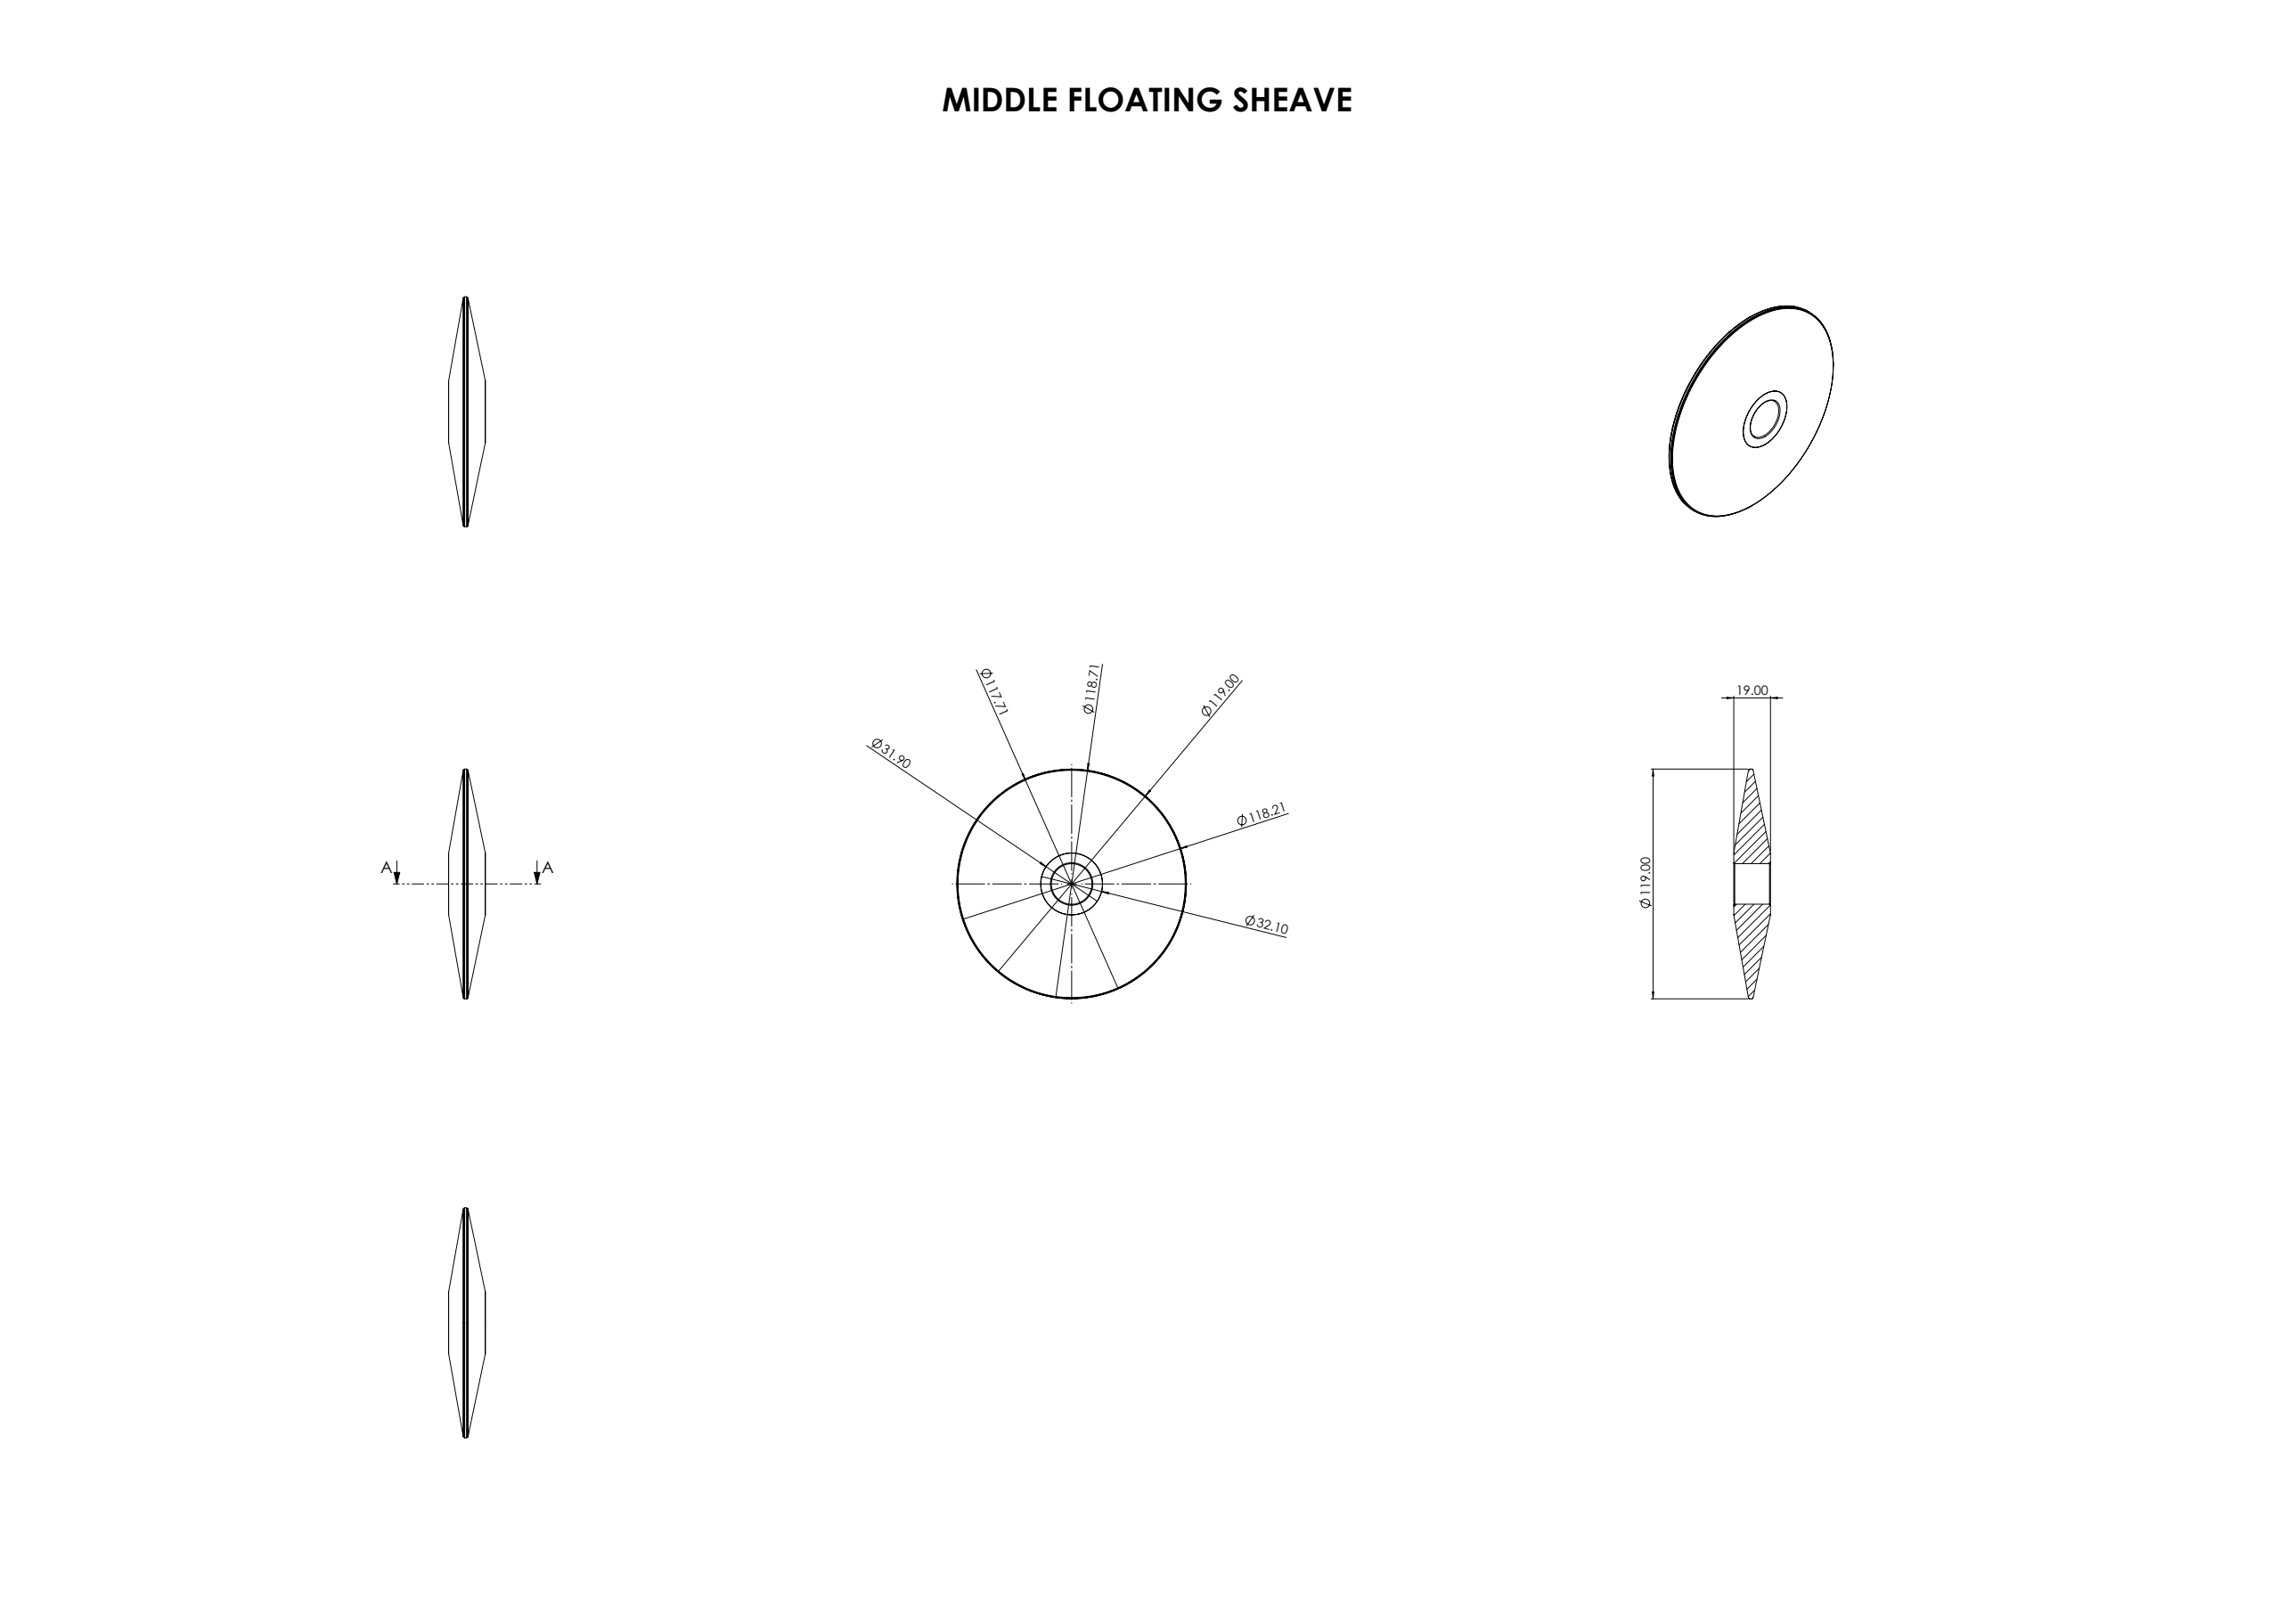
ISO-10303-21;
HEADER;
/* Generated by software containing ST-Developer
 * from STEP Tools, Inc. (www.steptools.com) 
 */

FILE_DESCRIPTION(
/* description */ (''),
/* implementation_level */ '2;1');

FILE_NAME(
/* name */ '02_Middle_Floating_Sheave.step',
/* time_stamp */ '2026-10-24T13:41:11-07:00',
/* author */ (''),
/* organization */ (''),
/* preprocessor_version */ 'ST-DEVELOPER v20.2',
/* originating_system */ 'Autodesk Translation Framework v15.15.0.0',
/* authorisation */ '');

FILE_SCHEMA (('AUTOMOTIVE_DESIGN { 1 0 10303 214 3 1 1 }'));
ENDSEC;

DATA;
#10=MECHANICAL_DESIGN_GEOMETRIC_PRESENTATION_REPRESENTATION('',(#122),#12813);
#81=CONICAL_SURFACE('',#4567,37.5,1.36447243276518);
#82=CONICAL_SURFACE('',#4576,59.25,0.785398163397448);
#83=CONICAL_SURFACE('',#4590,59.25,0.785398163397448);
#84=CONICAL_SURFACE('',#4597,37.5,1.39585880542621);
#102=SHAPE_REPRESENTATION_RELATIONSHIP('SRR','None',#12855,#112);
#112=ADVANCED_BREP_SHAPE_REPRESENTATION('',(#132),#12804);
#122=STYLED_ITEM('',(#12988),#132);
#132=MANIFOLD_SOLID_BREP('Body1',#4385);
#144=FACE_BOUND('',#632,.T.);
#145=FACE_BOUND('',#643,.T.);
#176=PLANE('',#4570);
#177=PLANE('',#4603);
#264=TOROIDAL_SURFACE('',#4562,15.9482352626124,0.5);
#265=TOROIDAL_SURFACE('',#4572,58.7517732660432,0.5);
#266=TOROIDAL_SURFACE('',#4579,59.,0.5);
#267=TOROIDAL_SURFACE('',#4586,59.,0.5);
#268=TOROIDAL_SURFACE('',#4593,58.7578429367487,0.5);
#269=TOROIDAL_SURFACE('',#4600,15.9561537431677,0.5);
#270=TOROIDAL_SURFACE('',#4605,11.,0.5);
#271=TOROIDAL_SURFACE('',#4612,11.,0.5);
#356=FACE_OUTER_BOUND('',#629,.T.);
#357=FACE_OUTER_BOUND('',#630,.T.);
#358=FACE_OUTER_BOUND('',#631,.T.);
#359=FACE_OUTER_BOUND('',#633,.T.);
#360=FACE_OUTER_BOUND('',#634,.T.);
#361=FACE_OUTER_BOUND('',#635,.T.);
#362=FACE_OUTER_BOUND('',#636,.T.);
#363=FACE_OUTER_BOUND('',#637,.T.);
#364=FACE_OUTER_BOUND('',#638,.T.);
#365=FACE_OUTER_BOUND('',#639,.T.);
#366=FACE_OUTER_BOUND('',#640,.T.);
#367=FACE_OUTER_BOUND('',#641,.T.);
#368=FACE_OUTER_BOUND('',#642,.T.);
#369=FACE_OUTER_BOUND('',#644,.T.);
#370=FACE_OUTER_BOUND('',#645,.T.);
#371=FACE_OUTER_BOUND('',#646,.T.);
#629=EDGE_LOOP('',(#2913,#2914,#2915,#2916,#2917));
#630=EDGE_LOOP('',(#2918,#2919,#2920,#2921,#2922,#2923));
#631=EDGE_LOOP('',(#2924));
#632=EDGE_LOOP('',(#2925));
#633=EDGE_LOOP('',(#2926,#2927,#2928,#2929,#2930,#2931));
#634=EDGE_LOOP('',(#2932,#2933,#2934,#2935,#2936,#2937));
#635=EDGE_LOOP('',(#2938,#2939,#2940,#2941,#2942,#2943));
#636=EDGE_LOOP('',(#2944,#2945,#2946,#2947,#2948,#2949));
#637=EDGE_LOOP('',(#2950,#2951,#2952,#2953,#2954,#2955));
#638=EDGE_LOOP('',(#2956,#2957,#2958,#2959,#2960,#2961));
#639=EDGE_LOOP('',(#2962,#2963,#2964,#2965,#2966,#2967));
#640=EDGE_LOOP('',(#2968,#2969,#2970,#2971,#2972,#2973));
#641=EDGE_LOOP('',(#2974,#2975,#2976,#2977,#2978));
#642=EDGE_LOOP('',(#2979));
#643=EDGE_LOOP('',(#2980));
#644=EDGE_LOOP('',(#2981,#2982,#2983,#2984,#2985));
#645=EDGE_LOOP('',(#2986,#2987,#2988,#2989,#2990,#2991));
#646=EDGE_LOOP('',(#2992,#2993,#2994,#2995,#2996));
#924=CIRCLE('',#4563,15.9482352626124);
#925=CIRCLE('',#4564,0.5);
#926=CIRCLE('',#4565,16.0506668396737);
#927=CIRCLE('',#4566,16.0506668396737);
#928=CIRCLE('',#4568,58.8542048431045);
#929=CIRCLE('',#4569,58.8542048431045);
#930=CIRCLE('',#4571,11.);
#931=CIRCLE('',#4573,0.5);
#932=CIRCLE('',#4574,59.1053266566364);
#933=CIRCLE('',#4575,59.1053266566364);
#934=CIRCLE('',#4577,59.3535533905933);
#935=CIRCLE('',#4578,59.3535533905933);
#936=CIRCLE('',#4580,0.5);
#937=CIRCLE('',#4581,59.5);
#938=CIRCLE('',#4582,59.5);
#939=CIRCLE('',#4584,59.5);
#940=CIRCLE('',#4585,59.5);
#941=CIRCLE('',#4587,0.5);
#942=CIRCLE('',#4588,59.3535533905933);
#943=CIRCLE('',#4589,59.3535533905933);
#944=CIRCLE('',#4591,59.111396327342);
#945=CIRCLE('',#4592,59.111396327342);
#946=CIRCLE('',#4594,0.5);
#947=CIRCLE('',#4595,58.8448662431924);
#948=CIRCLE('',#4596,58.8448662431924);
#949=CIRCLE('',#4598,16.0431770496114);
#950=CIRCLE('',#4599,16.0431770496114);
#951=CIRCLE('',#4601,0.5);
#952=CIRCLE('',#4602,15.9561537431677);
#953=CIRCLE('',#4604,11.);
#954=CIRCLE('',#4606,0.5);
#955=CIRCLE('',#4607,10.5);
#956=CIRCLE('',#4608,10.5);
#957=CIRCLE('',#4610,10.5);
#958=CIRCLE('',#4611,10.5);
#959=CIRCLE('',#4613,0.5);
#1139=LINE('',#7655,#1369);
#1140=LINE('',#7670,#1370);
#1141=LINE('',#7682,#1371);
#1142=LINE('',#7694,#1372);
#1143=LINE('',#7706,#1373);
#1144=LINE('',#7728,#1374);
#1369=VECTOR('',#5146,37.5);
#1370=VECTOR('',#5165,59.25);
#1371=VECTOR('',#5180,59.5);
#1372=VECTOR('',#5195,59.25);
#1373=VECTOR('',#5210,37.5);
#1374=VECTOR('',#5239,10.5);
#1789=VERTEX_POINT('',#7646);
#1790=VERTEX_POINT('',#7648);
#1791=VERTEX_POINT('',#7650);
#1792=VERTEX_POINT('',#7654);
#1793=VERTEX_POINT('',#7656);
#1794=VERTEX_POINT('',#7660);
#1795=VERTEX_POINT('',#7663);
#1796=VERTEX_POINT('',#7665);
#1797=VERTEX_POINT('',#7669);
#1798=VERTEX_POINT('',#7671);
#1799=VERTEX_POINT('',#7675);
#1800=VERTEX_POINT('',#7677);
#1801=VERTEX_POINT('',#7681);
#1802=VERTEX_POINT('',#7683);
#1803=VERTEX_POINT('',#7687);
#1804=VERTEX_POINT('',#7689);
#1805=VERTEX_POINT('',#7693);
#1806=VERTEX_POINT('',#7695);
#1807=VERTEX_POINT('',#7699);
#1808=VERTEX_POINT('',#7701);
#1809=VERTEX_POINT('',#7705);
#1810=VERTEX_POINT('',#7707);
#1811=VERTEX_POINT('',#7711);
#1812=VERTEX_POINT('',#7715);
#1813=VERTEX_POINT('',#7718);
#1814=VERTEX_POINT('',#7720);
#1815=VERTEX_POINT('',#7724);
#1816=VERTEX_POINT('',#7725);
#2209=EDGE_CURVE('',#1789,#1789,#924,.T.);
#2210=EDGE_CURVE('',#1789,#1790,#925,.T.);
#2211=EDGE_CURVE('',#1790,#1791,#926,.T.);
#2212=EDGE_CURVE('',#1791,#1790,#927,.T.);
#2213=EDGE_CURVE('',#1791,#1792,#1139,.T.);
#2214=EDGE_CURVE('',#1793,#1792,#928,.T.);
#2215=EDGE_CURVE('',#1792,#1793,#929,.T.);
#2216=EDGE_CURVE('',#1794,#1794,#930,.T.);
#2217=EDGE_CURVE('',#1793,#1795,#931,.T.);
#2218=EDGE_CURVE('',#1795,#1796,#932,.T.);
#2219=EDGE_CURVE('',#1796,#1795,#933,.T.);
#2220=EDGE_CURVE('',#1796,#1797,#1140,.T.);
#2221=EDGE_CURVE('',#1798,#1797,#934,.T.);
#2222=EDGE_CURVE('',#1797,#1798,#935,.T.);
#2223=EDGE_CURVE('',#1798,#1799,#936,.T.);
#2224=EDGE_CURVE('',#1799,#1800,#937,.T.);
#2225=EDGE_CURVE('',#1800,#1799,#938,.T.);
#2226=EDGE_CURVE('',#1800,#1801,#1141,.T.);
#2227=EDGE_CURVE('',#1802,#1801,#939,.T.);
#2228=EDGE_CURVE('',#1801,#1802,#940,.T.);
#2229=EDGE_CURVE('',#1802,#1803,#941,.T.);
#2230=EDGE_CURVE('',#1803,#1804,#942,.T.);
#2231=EDGE_CURVE('',#1804,#1803,#943,.T.);
#2232=EDGE_CURVE('',#1804,#1805,#1142,.T.);
#2233=EDGE_CURVE('',#1806,#1805,#944,.T.);
#2234=EDGE_CURVE('',#1805,#1806,#945,.T.);
#2235=EDGE_CURVE('',#1806,#1807,#946,.T.);
#2236=EDGE_CURVE('',#1807,#1808,#947,.T.);
#2237=EDGE_CURVE('',#1808,#1807,#948,.T.);
#2238=EDGE_CURVE('',#1808,#1809,#1143,.T.);
#2239=EDGE_CURVE('',#1810,#1809,#949,.T.);
#2240=EDGE_CURVE('',#1809,#1810,#950,.T.);
#2241=EDGE_CURVE('',#1810,#1811,#951,.T.);
#2242=EDGE_CURVE('',#1811,#1811,#952,.T.);
#2243=EDGE_CURVE('',#1812,#1812,#953,.T.);
#2244=EDGE_CURVE('',#1812,#1813,#954,.T.);
#2245=EDGE_CURVE('',#1813,#1814,#955,.T.);
#2246=EDGE_CURVE('',#1814,#1813,#956,.T.);
#2247=EDGE_CURVE('',#1815,#1816,#957,.T.);
#2248=EDGE_CURVE('',#1816,#1815,#958,.T.);
#2249=EDGE_CURVE('',#1816,#1814,#1144,.T.);
#2250=EDGE_CURVE('',#1815,#1794,#959,.T.);
#2913=ORIENTED_EDGE('',*,*,#2209,.T.);
#2914=ORIENTED_EDGE('',*,*,#2210,.T.);
#2915=ORIENTED_EDGE('',*,*,#2211,.T.);
#2916=ORIENTED_EDGE('',*,*,#2212,.T.);
#2917=ORIENTED_EDGE('',*,*,#2210,.F.);
#2918=ORIENTED_EDGE('',*,*,#2212,.F.);
#2919=ORIENTED_EDGE('',*,*,#2213,.T.);
#2920=ORIENTED_EDGE('',*,*,#2214,.F.);
#2921=ORIENTED_EDGE('',*,*,#2215,.F.);
#2922=ORIENTED_EDGE('',*,*,#2213,.F.);
#2923=ORIENTED_EDGE('',*,*,#2211,.F.);
#2924=ORIENTED_EDGE('',*,*,#2209,.F.);
#2925=ORIENTED_EDGE('',*,*,#2216,.F.);
#2926=ORIENTED_EDGE('',*,*,#2214,.T.);
#2927=ORIENTED_EDGE('',*,*,#2215,.T.);
#2928=ORIENTED_EDGE('',*,*,#2217,.T.);
#2929=ORIENTED_EDGE('',*,*,#2218,.T.);
#2930=ORIENTED_EDGE('',*,*,#2219,.T.);
#2931=ORIENTED_EDGE('',*,*,#2217,.F.);
#2932=ORIENTED_EDGE('',*,*,#2219,.F.);
#2933=ORIENTED_EDGE('',*,*,#2220,.T.);
#2934=ORIENTED_EDGE('',*,*,#2221,.F.);
#2935=ORIENTED_EDGE('',*,*,#2222,.F.);
#2936=ORIENTED_EDGE('',*,*,#2220,.F.);
#2937=ORIENTED_EDGE('',*,*,#2218,.F.);
#2938=ORIENTED_EDGE('',*,*,#2221,.T.);
#2939=ORIENTED_EDGE('',*,*,#2222,.T.);
#2940=ORIENTED_EDGE('',*,*,#2223,.T.);
#2941=ORIENTED_EDGE('',*,*,#2224,.T.);
#2942=ORIENTED_EDGE('',*,*,#2225,.T.);
#2943=ORIENTED_EDGE('',*,*,#2223,.F.);
#2944=ORIENTED_EDGE('',*,*,#2225,.F.);
#2945=ORIENTED_EDGE('',*,*,#2226,.T.);
#2946=ORIENTED_EDGE('',*,*,#2227,.F.);
#2947=ORIENTED_EDGE('',*,*,#2228,.F.);
#2948=ORIENTED_EDGE('',*,*,#2226,.F.);
#2949=ORIENTED_EDGE('',*,*,#2224,.F.);
#2950=ORIENTED_EDGE('',*,*,#2227,.T.);
#2951=ORIENTED_EDGE('',*,*,#2228,.T.);
#2952=ORIENTED_EDGE('',*,*,#2229,.T.);
#2953=ORIENTED_EDGE('',*,*,#2230,.T.);
#2954=ORIENTED_EDGE('',*,*,#2231,.T.);
#2955=ORIENTED_EDGE('',*,*,#2229,.F.);
#2956=ORIENTED_EDGE('',*,*,#2231,.F.);
#2957=ORIENTED_EDGE('',*,*,#2232,.T.);
#2958=ORIENTED_EDGE('',*,*,#2233,.F.);
#2959=ORIENTED_EDGE('',*,*,#2234,.F.);
#2960=ORIENTED_EDGE('',*,*,#2232,.F.);
#2961=ORIENTED_EDGE('',*,*,#2230,.F.);
#2962=ORIENTED_EDGE('',*,*,#2233,.T.);
#2963=ORIENTED_EDGE('',*,*,#2234,.T.);
#2964=ORIENTED_EDGE('',*,*,#2235,.T.);
#2965=ORIENTED_EDGE('',*,*,#2236,.T.);
#2966=ORIENTED_EDGE('',*,*,#2237,.T.);
#2967=ORIENTED_EDGE('',*,*,#2235,.F.);
#2968=ORIENTED_EDGE('',*,*,#2237,.F.);
#2969=ORIENTED_EDGE('',*,*,#2238,.T.);
#2970=ORIENTED_EDGE('',*,*,#2239,.F.);
#2971=ORIENTED_EDGE('',*,*,#2240,.F.);
#2972=ORIENTED_EDGE('',*,*,#2238,.F.);
#2973=ORIENTED_EDGE('',*,*,#2236,.F.);
#2974=ORIENTED_EDGE('',*,*,#2239,.T.);
#2975=ORIENTED_EDGE('',*,*,#2240,.T.);
#2976=ORIENTED_EDGE('',*,*,#2241,.T.);
#2977=ORIENTED_EDGE('',*,*,#2242,.T.);
#2978=ORIENTED_EDGE('',*,*,#2241,.F.);
#2979=ORIENTED_EDGE('',*,*,#2242,.F.);
#2980=ORIENTED_EDGE('',*,*,#2243,.F.);
#2981=ORIENTED_EDGE('',*,*,#2243,.T.);
#2982=ORIENTED_EDGE('',*,*,#2244,.T.);
#2983=ORIENTED_EDGE('',*,*,#2245,.T.);
#2984=ORIENTED_EDGE('',*,*,#2246,.T.);
#2985=ORIENTED_EDGE('',*,*,#2244,.F.);
#2986=ORIENTED_EDGE('',*,*,#2247,.F.);
#2987=ORIENTED_EDGE('',*,*,#2248,.F.);
#2988=ORIENTED_EDGE('',*,*,#2249,.T.);
#2989=ORIENTED_EDGE('',*,*,#2245,.F.);
#2990=ORIENTED_EDGE('',*,*,#2246,.F.);
#2991=ORIENTED_EDGE('',*,*,#2249,.F.);
#2992=ORIENTED_EDGE('',*,*,#2247,.T.);
#2993=ORIENTED_EDGE('',*,*,#2248,.T.);
#2994=ORIENTED_EDGE('',*,*,#2250,.T.);
#2995=ORIENTED_EDGE('',*,*,#2216,.T.);
#2996=ORIENTED_EDGE('',*,*,#2250,.F.);
#4038=CYLINDRICAL_SURFACE('',#4583,59.5);
#4039=CYLINDRICAL_SURFACE('',#4609,10.5);
#4146=ADVANCED_FACE('',(#356),#264,.T.);
#4147=ADVANCED_FACE('',(#357),#81,.T.);
#4148=ADVANCED_FACE('',(#358,#144),#176,.T.);
#4149=ADVANCED_FACE('',(#359),#265,.T.);
#4150=ADVANCED_FACE('',(#360),#82,.T.);
#4151=ADVANCED_FACE('',(#361),#266,.T.);
#4152=ADVANCED_FACE('',(#362),#4038,.T.);
#4153=ADVANCED_FACE('',(#363),#267,.T.);
#4154=ADVANCED_FACE('',(#364),#83,.T.);
#4155=ADVANCED_FACE('',(#365),#268,.T.);
#4156=ADVANCED_FACE('',(#366),#84,.T.);
#4157=ADVANCED_FACE('',(#367),#269,.T.);
#4158=ADVANCED_FACE('',(#368,#145),#177,.T.);
#4159=ADVANCED_FACE('',(#369),#270,.T.);
#4160=ADVANCED_FACE('',(#370),#4039,.F.);
#4161=ADVANCED_FACE('',(#371),#271,.T.);
#4385=CLOSED_SHELL('',(#4146,#4147,#4148,#4149,#4150,#4151,#4152,#4153,
#4154,#4155,#4156,#4157,#4158,#4159,#4160,#4161));
#4561=AXIS2_PLACEMENT_3D('',#7644,#5132,#5133);
#4562=AXIS2_PLACEMENT_3D('',#7645,#5134,#5135);
#4563=AXIS2_PLACEMENT_3D('',#7647,#5136,#5137);
#4564=AXIS2_PLACEMENT_3D('',#7649,#5138,#5139);
#4565=AXIS2_PLACEMENT_3D('',#7651,#5140,#5141);
#4566=AXIS2_PLACEMENT_3D('',#7652,#5142,#5143);
#4567=AXIS2_PLACEMENT_3D('',#7653,#5144,#5145);
#4568=AXIS2_PLACEMENT_3D('',#7657,#5147,#5148);
#4569=AXIS2_PLACEMENT_3D('',#7658,#5149,#5150);
#4570=AXIS2_PLACEMENT_3D('',#7659,#5151,#5152);
#4571=AXIS2_PLACEMENT_3D('',#7661,#5153,#5154);
#4572=AXIS2_PLACEMENT_3D('',#7662,#5155,#5156);
#4573=AXIS2_PLACEMENT_3D('',#7664,#5157,#5158);
#4574=AXIS2_PLACEMENT_3D('',#7666,#5159,#5160);
#4575=AXIS2_PLACEMENT_3D('',#7667,#5161,#5162);
#4576=AXIS2_PLACEMENT_3D('',#7668,#5163,#5164);
#4577=AXIS2_PLACEMENT_3D('',#7672,#5166,#5167);
#4578=AXIS2_PLACEMENT_3D('',#7673,#5168,#5169);
#4579=AXIS2_PLACEMENT_3D('',#7674,#5170,#5171);
#4580=AXIS2_PLACEMENT_3D('',#7676,#5172,#5173);
#4581=AXIS2_PLACEMENT_3D('',#7678,#5174,#5175);
#4582=AXIS2_PLACEMENT_3D('',#7679,#5176,#5177);
#4583=AXIS2_PLACEMENT_3D('',#7680,#5178,#5179);
#4584=AXIS2_PLACEMENT_3D('',#7684,#5181,#5182);
#4585=AXIS2_PLACEMENT_3D('',#7685,#5183,#5184);
#4586=AXIS2_PLACEMENT_3D('',#7686,#5185,#5186);
#4587=AXIS2_PLACEMENT_3D('',#7688,#5187,#5188);
#4588=AXIS2_PLACEMENT_3D('',#7690,#5189,#5190);
#4589=AXIS2_PLACEMENT_3D('',#7691,#5191,#5192);
#4590=AXIS2_PLACEMENT_3D('',#7692,#5193,#5194);
#4591=AXIS2_PLACEMENT_3D('',#7696,#5196,#5197);
#4592=AXIS2_PLACEMENT_3D('',#7697,#5198,#5199);
#4593=AXIS2_PLACEMENT_3D('',#7698,#5200,#5201);
#4594=AXIS2_PLACEMENT_3D('',#7700,#5202,#5203);
#4595=AXIS2_PLACEMENT_3D('',#7702,#5204,#5205);
#4596=AXIS2_PLACEMENT_3D('',#7703,#5206,#5207);
#4597=AXIS2_PLACEMENT_3D('',#7704,#5208,#5209);
#4598=AXIS2_PLACEMENT_3D('',#7708,#5211,#5212);
#4599=AXIS2_PLACEMENT_3D('',#7709,#5213,#5214);
#4600=AXIS2_PLACEMENT_3D('',#7710,#5215,#5216);
#4601=AXIS2_PLACEMENT_3D('',#7712,#5217,#5218);
#4602=AXIS2_PLACEMENT_3D('',#7713,#5219,#5220);
#4603=AXIS2_PLACEMENT_3D('',#7714,#5221,#5222);
#4604=AXIS2_PLACEMENT_3D('',#7716,#5223,#5224);
#4605=AXIS2_PLACEMENT_3D('',#7717,#5225,#5226);
#4606=AXIS2_PLACEMENT_3D('',#7719,#5227,#5228);
#4607=AXIS2_PLACEMENT_3D('',#7721,#5229,#5230);
#4608=AXIS2_PLACEMENT_3D('',#7722,#5231,#5232);
#4609=AXIS2_PLACEMENT_3D('',#7723,#5233,#5234);
#4610=AXIS2_PLACEMENT_3D('',#7726,#5235,#5236);
#4611=AXIS2_PLACEMENT_3D('',#7727,#5237,#5238);
#4612=AXIS2_PLACEMENT_3D('',#7729,#5240,#5241);
#4613=AXIS2_PLACEMENT_3D('',#7730,#5242,#5243);
#5132=DIRECTION('axis',(0.,0.,1.));
#5133=DIRECTION('refdir',(1.,0.,0.));
#5134=DIRECTION('center_axis',(1.,0.,0.));
#5135=DIRECTION('ref_axis',(0.,0.,-1.));
#5136=DIRECTION('center_axis',(-1.,0.,0.));
#5137=DIRECTION('ref_axis',(0.,-1.,1.83697019872103E-16));
#5138=DIRECTION('center_axis',(0.,-1.,-1.22464679914735E-16));
#5139=DIRECTION('ref_axis',(0.,-1.22464679914735E-16,1.));
#5140=DIRECTION('center_axis',(1.,0.,0.));
#5141=DIRECTION('ref_axis',(0.,-1.,3.06161699786838E-17));
#5142=DIRECTION('center_axis',(1.,0.,0.));
#5143=DIRECTION('ref_axis',(0.,-1.,3.06161699786838E-17));
#5144=DIRECTION('center_axis',(-1.,0.,0.));
#5145=DIRECTION('ref_axis',(0.,1.,0.));
#5146=DIRECTION('',(-0.204863154122693,-0.978790625252869,-1.19867280625136E-16));
#5147=DIRECTION('center_axis',(-1.,0.,0.));
#5148=DIRECTION('ref_axis',(0.,-1.,3.06161699786838E-17));
#5149=DIRECTION('center_axis',(-1.,0.,0.));
#5150=DIRECTION('ref_axis',(0.,-1.,3.06161699786838E-17));
#5151=DIRECTION('center_axis',(1.,0.,0.));
#5152=DIRECTION('ref_axis',(0.,0.,-1.));
#5153=DIRECTION('center_axis',(1.,0.,0.));
#5154=DIRECTION('ref_axis',(0.,-1.,1.83697019872103E-16));
#5155=DIRECTION('center_axis',(1.,0.,0.));
#5156=DIRECTION('ref_axis',(0.,0.,-1.));
#5157=DIRECTION('center_axis',(0.,-1.,-1.22464679914735E-16));
#5158=DIRECTION('ref_axis',(0.,-1.22464679914735E-16,1.));
#5159=DIRECTION('center_axis',(1.,0.,0.));
#5160=DIRECTION('ref_axis',(0.,-1.,3.06161699786838E-17));
#5161=DIRECTION('center_axis',(1.,0.,0.));
#5162=DIRECTION('ref_axis',(0.,-1.,3.06161699786838E-17));
#5163=DIRECTION('center_axis',(-1.,0.,0.));
#5164=DIRECTION('ref_axis',(0.,1.,0.));
#5165=DIRECTION('',(-0.707106781186547,-0.707106781186547,-8.65956056235494E-17));
#5166=DIRECTION('center_axis',(-1.,0.,0.));
#5167=DIRECTION('ref_axis',(0.,-1.,3.06161699786838E-17));
#5168=DIRECTION('center_axis',(-1.,0.,0.));
#5169=DIRECTION('ref_axis',(0.,-1.,3.06161699786838E-17));
#5170=DIRECTION('center_axis',(1.,0.,0.));
#5171=DIRECTION('ref_axis',(0.,0.,-1.));
#5172=DIRECTION('center_axis',(0.,-1.,-1.22464679914735E-16));
#5173=DIRECTION('ref_axis',(0.,-1.22464679914735E-16,1.));
#5174=DIRECTION('center_axis',(1.,0.,0.));
#5175=DIRECTION('ref_axis',(0.,-1.,1.83697019872103E-16));
#5176=DIRECTION('center_axis',(1.,0.,0.));
#5177=DIRECTION('ref_axis',(0.,-1.,1.83697019872103E-16));
#5178=DIRECTION('center_axis',(1.,0.,0.));
#5179=DIRECTION('ref_axis',(0.,1.,0.));
#5180=DIRECTION('',(-1.,0.,0.));
#5181=DIRECTION('center_axis',(-1.,0.,0.));
#5182=DIRECTION('ref_axis',(0.,-1.,1.83697019872103E-16));
#5183=DIRECTION('center_axis',(-1.,0.,0.));
#5184=DIRECTION('ref_axis',(0.,-1.,1.83697019872103E-16));
#5185=DIRECTION('center_axis',(1.,0.,0.));
#5186=DIRECTION('ref_axis',(0.,0.,-1.));
#5187=DIRECTION('center_axis',(0.,-1.,-1.22464679914735E-16));
#5188=DIRECTION('ref_axis',(0.,-1.22464679914735E-16,1.));
#5189=DIRECTION('center_axis',(1.,0.,0.));
#5190=DIRECTION('ref_axis',(0.,-1.,3.06161699786838E-17));
#5191=DIRECTION('center_axis',(1.,0.,0.));
#5192=DIRECTION('ref_axis',(0.,-1.,3.06161699786838E-17));
#5193=DIRECTION('center_axis',(1.,0.,0.));
#5194=DIRECTION('ref_axis',(0.,1.,0.));
#5195=DIRECTION('',(-0.707106781186547,0.707106781186547,8.65956056235494E-17));
#5196=DIRECTION('center_axis',(-1.,0.,0.));
#5197=DIRECTION('ref_axis',(0.,-1.,3.06161699786838E-17));
#5198=DIRECTION('center_axis',(-1.,0.,0.));
#5199=DIRECTION('ref_axis',(0.,-1.,3.06161699786838E-17));
#5200=DIRECTION('center_axis',(1.,0.,0.));
#5201=DIRECTION('ref_axis',(0.,0.,-1.));
#5202=DIRECTION('center_axis',(0.,-1.,-1.22464679914735E-16));
#5203=DIRECTION('ref_axis',(0.,-1.22464679914735E-16,1.));
#5204=DIRECTION('center_axis',(1.,0.,0.));
#5205=DIRECTION('ref_axis',(0.,-1.,3.06161699786838E-17));
#5206=DIRECTION('center_axis',(1.,0.,0.));
#5207=DIRECTION('ref_axis',(0.,-1.,3.06161699786838E-17));
#5208=DIRECTION('center_axis',(1.,0.,0.));
#5209=DIRECTION('ref_axis',(0.,1.,0.));
#5210=DIRECTION('',(-0.174046612887447,0.984737415021084,1.20595552330621E-16));
#5211=DIRECTION('center_axis',(-1.,0.,0.));
#5212=DIRECTION('ref_axis',(0.,-1.,3.06161699786838E-17));
#5213=DIRECTION('center_axis',(-1.,0.,0.));
#5214=DIRECTION('ref_axis',(0.,-1.,3.06161699786838E-17));
#5215=DIRECTION('center_axis',(1.,0.,0.));
#5216=DIRECTION('ref_axis',(0.,0.,-1.));
#5217=DIRECTION('center_axis',(0.,-1.,-1.22464679914735E-16));
#5218=DIRECTION('ref_axis',(0.,-1.22464679914735E-16,1.));
#5219=DIRECTION('center_axis',(1.,0.,0.));
#5220=DIRECTION('ref_axis',(0.,-1.,1.83697019872103E-16));
#5221=DIRECTION('center_axis',(-1.,0.,0.));
#5222=DIRECTION('ref_axis',(0.,0.,1.));
#5223=DIRECTION('center_axis',(-1.,0.,0.));
#5224=DIRECTION('ref_axis',(0.,-1.,1.83697019872103E-16));
#5225=DIRECTION('center_axis',(1.,0.,0.));
#5226=DIRECTION('ref_axis',(0.,0.,-1.));
#5227=DIRECTION('center_axis',(0.,-1.,-1.22464679914735E-16));
#5228=DIRECTION('ref_axis',(0.,-1.22464679914735E-16,1.));
#5229=DIRECTION('center_axis',(1.,0.,0.));
#5230=DIRECTION('ref_axis',(0.,-1.,1.83697019872103E-16));
#5231=DIRECTION('center_axis',(1.,0.,0.));
#5232=DIRECTION('ref_axis',(0.,-1.,1.83697019872103E-16));
#5233=DIRECTION('center_axis',(1.,0.,0.));
#5234=DIRECTION('ref_axis',(0.,1.,0.));
#5235=DIRECTION('center_axis',(-1.,0.,0.));
#5236=DIRECTION('ref_axis',(0.,-1.,1.83697019872103E-16));
#5237=DIRECTION('center_axis',(-1.,0.,0.));
#5238=DIRECTION('ref_axis',(0.,-1.,1.83697019872103E-16));
#5239=DIRECTION('',(-1.,0.,0.));
#5240=DIRECTION('center_axis',(1.,0.,0.));
#5241=DIRECTION('ref_axis',(0.,0.,-1.));
#5242=DIRECTION('center_axis',(0.,-1.,-1.22464679914735E-16));
#5243=DIRECTION('ref_axis',(0.,-1.22464679914735E-16,1.));
#7644=CARTESIAN_POINT('',(0.,0.,0.));
#7645=CARTESIAN_POINT('Origin',(33.5,0.,0.));
#7646=CARTESIAN_POINT('',(34.,-1.95309552664072E-15,15.9482352626124));
#7647=CARTESIAN_POINT('Origin',(34.,0.,0.));
#7648=CARTESIAN_POINT('',(33.9893953126264,-1.9656397769387E-15,16.0506668396737));
#7649=CARTESIAN_POINT('Origin',(33.5,-1.95309552664072E-15,15.9482352626124));
#7650=CARTESIAN_POINT('',(33.9893953126264,-16.0506668396737,-1.96563977693869E-15));
#7651=CARTESIAN_POINT('Origin',(33.9893953126264,0.,-2.45704972117337E-15));
#7652=CARTESIAN_POINT('Origin',(33.9893953126264,0.,-2.45704972117337E-15));
#7653=CARTESIAN_POINT('Origin',(29.5,0.,0.));
#7654=CARTESIAN_POINT('',(25.0305152653967,-58.8542048431045,-7.20756135774706E-15));
#7655=CARTESIAN_POINT('',(29.5,-37.5,-4.59242549680258E-15));
#7656=CARTESIAN_POINT('',(25.0305152653967,-7.20756135774706E-15,58.8542048431045));
#7657=CARTESIAN_POINT('Origin',(25.0305152653967,0.,-9.00945169718383E-15));
#7658=CARTESIAN_POINT('Origin',(25.0305152653967,0.,-9.00945169718383E-15));
#7659=CARTESIAN_POINT('Origin',(34.,10.5,0.));
#7660=CARTESIAN_POINT('',(34.,-1.34711147906209E-15,11.));
#7661=CARTESIAN_POINT('Origin',(34.,0.,0.));
#7662=CARTESIAN_POINT('Origin',(24.5411199527703,0.,0.));
#7663=CARTESIAN_POINT('',(24.8946733433636,-7.23831491026085E-15,59.1053266566364));
#7664=CARTESIAN_POINT('Origin',(24.5411199527703,-7.19501710744908E-15,
58.7517732660432));
#7665=CARTESIAN_POINT('',(24.8946733433636,-59.1053266566364,-7.23831491026085E-15));
#7666=CARTESIAN_POINT('Origin',(24.8946733433636,0.,-9.04789363782607E-15));
#7667=CARTESIAN_POINT('Origin',(24.8946733433636,0.,-9.04789363782607E-15));
#7668=CARTESIAN_POINT('Origin',(24.75,0.,0.));
#7669=CARTESIAN_POINT('',(24.6464466094067,-59.3535533905933,-7.26871391778116E-15));
#7670=CARTESIAN_POINT('',(24.75,-59.25,-7.25603228494807E-15));
#7671=CARTESIAN_POINT('',(24.6464466094067,-7.26871391778116E-15,59.3535533905933));
#7672=CARTESIAN_POINT('Origin',(24.6464466094067,0.,-9.08589239722645E-15));
#7673=CARTESIAN_POINT('Origin',(24.6464466094067,0.,-9.08589239722645E-15));
#7674=CARTESIAN_POINT('Origin',(24.2928932188135,0.,0.));
#7675=CARTESIAN_POINT('',(24.2928932188135,-7.28664845492675E-15,59.5));
#7676=CARTESIAN_POINT('Origin',(24.2928932188135,-7.22541611496938E-15,
59.));
#7677=CARTESIAN_POINT('',(24.2928932188135,-59.5,-7.28664845492675E-15));
#7678=CARTESIAN_POINT('Origin',(24.2928932188135,0.,0.));
#7679=CARTESIAN_POINT('Origin',(24.2928932188135,0.,0.));
#7680=CARTESIAN_POINT('Origin',(23.8,0.,0.));
#7681=CARTESIAN_POINT('',(23.3071067811865,-59.5,-7.28664845492675E-15));
#7682=CARTESIAN_POINT('',(23.8,-59.5,-7.28664845492675E-15));
#7683=CARTESIAN_POINT('',(23.3071067811865,-7.28664845492675E-15,59.5));
#7684=CARTESIAN_POINT('Origin',(23.3071067811865,0.,0.));
#7685=CARTESIAN_POINT('Origin',(23.3071067811865,0.,0.));
#7686=CARTESIAN_POINT('Origin',(23.3071067811865,0.,0.));
#7687=CARTESIAN_POINT('',(22.9535533905933,-7.26871391778116E-15,59.3535533905933));
#7688=CARTESIAN_POINT('Origin',(23.3071067811865,-7.22541611496938E-15,
59.));
#7689=CARTESIAN_POINT('',(22.9535533905933,-59.3535533905933,-7.26871391778116E-15));
#7690=CARTESIAN_POINT('Origin',(22.9535533905933,0.,-9.08589239722645E-15));
#7691=CARTESIAN_POINT('Origin',(22.9535533905933,0.,-9.08589239722645E-15));
#7692=CARTESIAN_POINT('Origin',(22.85,0.,0.));
#7693=CARTESIAN_POINT('',(22.711396327342,-59.111396327342,-7.239058230541E-15));
#7694=CARTESIAN_POINT('',(22.85,-59.25,-7.25603228494807E-15));
#7695=CARTESIAN_POINT('',(22.711396327342,-7.239058230541E-15,59.111396327342));
#7696=CARTESIAN_POINT('Origin',(22.711396327342,0.,-9.04882278817625E-15));
#7697=CARTESIAN_POINT('Origin',(22.711396327342,0.,-9.04882278817625E-15));
#7698=CARTESIAN_POINT('Origin',(23.0649497179352,0.,0.));
#7699=CARTESIAN_POINT('',(22.5725810104247,-7.20641770909798E-15,58.8448662431924));
#7700=CARTESIAN_POINT('Origin',(23.0649497179352,-7.19576042772922E-15,
58.7578429367487));
#7701=CARTESIAN_POINT('',(22.5725810104247,-58.8448662431925,-7.20641770909798E-15));
#7702=CARTESIAN_POINT('Origin',(22.5725810104247,0.,-9.00802213637247E-15));
#7703=CARTESIAN_POINT('Origin',(22.5725810104247,0.,-9.00802213637247E-15));
#7704=CARTESIAN_POINT('Origin',(18.8,0.,0.));
#7705=CARTESIAN_POINT('',(15.0076312924895,-16.0431770496114,-1.96472254219609E-15));
#7706=CARTESIAN_POINT('',(18.8,-37.5,-4.59242549680258E-15));
#7707=CARTESIAN_POINT('',(15.0076312924895,-1.96472254219609E-15,16.0431770496114));
#7708=CARTESIAN_POINT('Origin',(15.0076312924895,0.,-2.45590317774511E-15));
#7709=CARTESIAN_POINT('Origin',(15.0076312924895,0.,-2.45590317774511E-15));
#7710=CARTESIAN_POINT('Origin',(15.5,0.,0.));
#7711=CARTESIAN_POINT('',(15.,-1.95406526082734E-15,15.9561537431677));
#7712=CARTESIAN_POINT('Origin',(15.5,-1.95406526082734E-15,15.9561537431677));
#7713=CARTESIAN_POINT('Origin',(15.,0.,0.));
#7714=CARTESIAN_POINT('Origin',(15.,16.,0.));
#7715=CARTESIAN_POINT('',(15.,-1.34711147906209E-15,11.));
#7716=CARTESIAN_POINT('Origin',(15.,0.,0.));
#7717=CARTESIAN_POINT('Origin',(15.5,0.,0.));
#7718=CARTESIAN_POINT('',(15.5,-1.28587913910472E-15,10.5));
#7719=CARTESIAN_POINT('Origin',(15.5,-1.34711147906209E-15,11.));
#7720=CARTESIAN_POINT('',(15.5,-10.5,-1.28587913910472E-15));
#7721=CARTESIAN_POINT('Origin',(15.5,0.,0.));
#7722=CARTESIAN_POINT('Origin',(15.5,0.,0.));
#7723=CARTESIAN_POINT('Origin',(24.5,0.,0.));
#7724=CARTESIAN_POINT('',(33.5,-1.28587913910472E-15,10.5));
#7725=CARTESIAN_POINT('',(33.5,-10.5,-1.28587913910472E-15));
#7726=CARTESIAN_POINT('Origin',(33.5,0.,0.));
#7727=CARTESIAN_POINT('Origin',(33.5,0.,0.));
#7728=CARTESIAN_POINT('',(24.5,-10.5,-1.28587913910472E-15));
#7729=CARTESIAN_POINT('Origin',(33.5,0.,0.));
#7730=CARTESIAN_POINT('Origin',(33.5,-1.34711147906209E-15,11.));
#12792=UNCERTAINTY_MEASURE_WITH_UNIT(LENGTH_MEASURE(0.01),#12814,
'DISTANCE_ACCURACY_VALUE',
'Maximum model space distance between geometric entities at asserted c
onnectivities');
#12801=UNCERTAINTY_MEASURE_WITH_UNIT(LENGTH_MEASURE(0.01),#12814,
'DISTANCE_ACCURACY_VALUE',
'Maximum model space distance between geometric entities at asserted c
onnectivities');
#12804=(
GEOMETRIC_REPRESENTATION_CONTEXT(3)
GLOBAL_UNCERTAINTY_ASSIGNED_CONTEXT((#12792))
GLOBAL_UNIT_ASSIGNED_CONTEXT((#12814,#12816,#12817))
REPRESENTATION_CONTEXT('','3D')
);
#12813=(
GEOMETRIC_REPRESENTATION_CONTEXT(3)
GLOBAL_UNCERTAINTY_ASSIGNED_CONTEXT((#12801))
GLOBAL_UNIT_ASSIGNED_CONTEXT((#12814,#12816,#12817))
REPRESENTATION_CONTEXT('','3D')
);
#12814=(
LENGTH_UNIT()
NAMED_UNIT(*)
SI_UNIT(.MILLI.,.METRE.)
);
#12816=(
NAMED_UNIT(*)
PLANE_ANGLE_UNIT()
SI_UNIT($,.RADIAN.)
);
#12817=(
NAMED_UNIT(*)
SI_UNIT($,.STERADIAN.)
SOLID_ANGLE_UNIT()
);
#12820=SHAPE_DEFINITION_REPRESENTATION(#12831,#12855);
#12831=PRODUCT_DEFINITION_SHAPE('',$,#12867);
#12855=SHAPE_REPRESENTATION('',(#4561),#12804);
#12864=PRODUCT_DEFINITION_CONTEXT('part definition',#12899,'design');
#12867=PRODUCT_DEFINITION('2026-10-11-12-17-35-115',
'02_Middle_Floating_Sheave',#12878,#12864);
#12878=PRODUCT_DEFINITION_FORMATION('',$,#12903);
#12899=APPLICATION_CONTEXT(
'Core Data for Automotive Mechanical Design Process');
#12900=PRODUCT_CONTEXT('part definition',#12899,'mechanical');
#12903=PRODUCT('2026-10-11-12-17-35-115','02_Middle_Floating_Sheave',$,
(#12900));
#12982=COLOUR_RGB('Off White',0.89,0.88,0.83);
#12983=FILL_AREA_STYLE_COLOUR('',#12982);
#12984=FILL_AREA_STYLE('',(#12983));
#12985=SURFACE_STYLE_FILL_AREA(#12984);
#12986=SURFACE_SIDE_STYLE('',(#12985));
#12987=SURFACE_STYLE_USAGE(.BOTH.,#12986);
#12988=PRESENTATION_STYLE_ASSIGNMENT((#12987));
ENDSEC;
END-ISO-10303-21;
